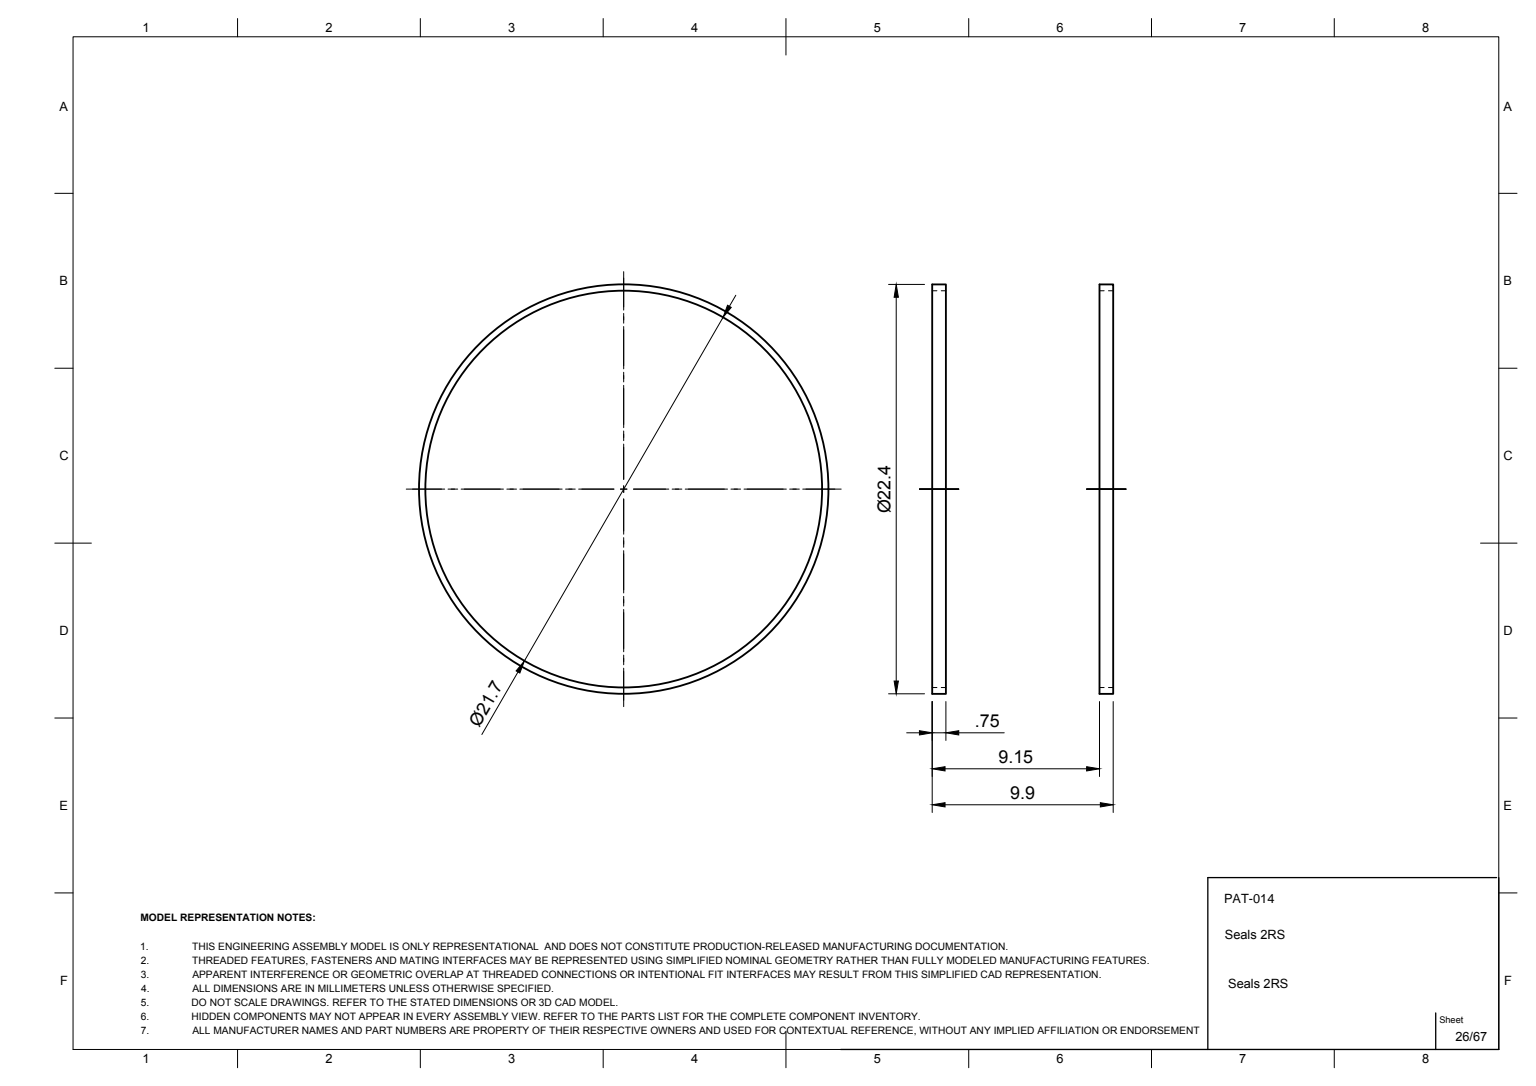
ISO-10303-21;
HEADER;
/* Generated by software containing ST-Developer
 * from STEP Tools, Inc. (www.steptools.com) 
 */

FILE_DESCRIPTION(
/* description */ ('Bin tilter linkage'),
/* implementation_level */ '2;1');

FILE_NAME(
/* name */ 'Seals 2RS.step',
/* time_stamp */ '2026-10-28T03:26:24-07:00',
/* author */ (''),
/* organization */ (''),
/* preprocessor_version */ 'ST-DEVELOPER v20.2',
/* originating_system */ 'Autodesk Translation Framework v15.17.0.0',
/* authorisation */ '');

FILE_SCHEMA (('AUTOMOTIVE_DESIGN { 1 0 10303 214 3 1 1 }'));
ENDSEC;

DATA;
#10=MECHANICAL_DESIGN_GEOMETRIC_PRESENTATION_REPRESENTATION('',(#944,#945),#23728);
#726=SHAPE_REPRESENTATION_RELATIONSHIP('SRR','None',#24193,#832);
#832=ADVANCED_BREP_SHAPE_REPRESENTATION('',(#1057,#1058),#23693);
#944=STYLED_ITEM('',(#24765),#1057);
#945=STYLED_ITEM('',(#24765),#1058);
#1057=MANIFOLD_SOLID_BREP('Body1',#12475);
#1058=MANIFOLD_SOLID_BREP('Body2',#12476);
#1391=FACE_BOUND('',#3517,.T.);
#1392=FACE_BOUND('',#3520,.T.);
#1393=FACE_BOUND('',#3523,.T.);
#1394=FACE_BOUND('',#3526,.T.);
#1749=PLANE('',#14880);
#1750=PLANE('',#14885);
#1751=PLANE('',#14888);
#1752=PLANE('',#14893);
#2435=FACE_OUTER_BOUND('',#3516,.T.);
#2436=FACE_OUTER_BOUND('',#3518,.T.);
#2437=FACE_OUTER_BOUND('',#3519,.T.);
#2438=FACE_OUTER_BOUND('',#3521,.T.);
#2439=FACE_OUTER_BOUND('',#3522,.T.);
#2440=FACE_OUTER_BOUND('',#3524,.T.);
#2441=FACE_OUTER_BOUND('',#3525,.T.);
#2442=FACE_OUTER_BOUND('',#3527,.T.);
#3516=EDGE_LOOP('',(#10387));
#3517=EDGE_LOOP('',(#10388));
#3518=EDGE_LOOP('',(#10389,#10390,#10391,#10392));
#3519=EDGE_LOOP('',(#10393));
#3520=EDGE_LOOP('',(#10394));
#3521=EDGE_LOOP('',(#10395,#10396,#10397,#10398));
#3522=EDGE_LOOP('',(#10399));
#3523=EDGE_LOOP('',(#10400));
#3524=EDGE_LOOP('',(#10401,#10402,#10403,#10404));
#3525=EDGE_LOOP('',(#10405));
#3526=EDGE_LOOP('',(#10406));
#3527=EDGE_LOOP('',(#10407,#10408,#10409,#10410));
#4265=LINE('',#22359,#4940);
#4266=LINE('',#22364,#4941);
#4267=LINE('',#22373,#4942);
#4268=LINE('',#22378,#4943);
#4940=VECTOR('',#18308,1.119765);
#4941=VECTOR('',#18315,1.085235);
#4942=VECTOR('',#18326,1.119765);
#4943=VECTOR('',#18333,1.085235);
#5776=CIRCLE('',#14881,1.119765);
#5777=CIRCLE('',#14882,1.085235);
#5778=CIRCLE('',#14884,1.119765);
#5779=CIRCLE('',#14886,1.085235);
#5780=CIRCLE('',#14889,1.119765);
#5781=CIRCLE('',#14890,1.085235);
#5782=CIRCLE('',#14892,1.119765);
#5783=CIRCLE('',#14894,1.085235);
#6635=VERTEX_POINT('',#22352);
#6636=VERTEX_POINT('',#22354);
#6637=VERTEX_POINT('',#22357);
#6638=VERTEX_POINT('',#22361);
#6639=VERTEX_POINT('',#22366);
#6640=VERTEX_POINT('',#22368);
#6641=VERTEX_POINT('',#22371);
#6642=VERTEX_POINT('',#22375);
#7933=EDGE_CURVE('',#6635,#6635,#5776,.T.);
#7934=EDGE_CURVE('',#6636,#6636,#5777,.T.);
#7935=EDGE_CURVE('',#6637,#6637,#5778,.T.);
#7936=EDGE_CURVE('',#6637,#6635,#4265,.T.);
#7937=EDGE_CURVE('',#6638,#6638,#5779,.T.);
#7938=EDGE_CURVE('',#6638,#6636,#4266,.T.);
#7939=EDGE_CURVE('',#6639,#6639,#5780,.T.);
#7940=EDGE_CURVE('',#6640,#6640,#5781,.T.);
#7941=EDGE_CURVE('',#6641,#6641,#5782,.T.);
#7942=EDGE_CURVE('',#6641,#6639,#4267,.T.);
#7943=EDGE_CURVE('',#6642,#6642,#5783,.T.);
#7944=EDGE_CURVE('',#6642,#6640,#4268,.T.);
#10387=ORIENTED_EDGE('',*,*,#7933,.F.);
#10388=ORIENTED_EDGE('',*,*,#7934,.T.);
#10389=ORIENTED_EDGE('',*,*,#7935,.F.);
#10390=ORIENTED_EDGE('',*,*,#7936,.T.);
#10391=ORIENTED_EDGE('',*,*,#7933,.T.);
#10392=ORIENTED_EDGE('',*,*,#7936,.F.);
#10393=ORIENTED_EDGE('',*,*,#7935,.T.);
#10394=ORIENTED_EDGE('',*,*,#7937,.F.);
#10395=ORIENTED_EDGE('',*,*,#7937,.T.);
#10396=ORIENTED_EDGE('',*,*,#7938,.T.);
#10397=ORIENTED_EDGE('',*,*,#7934,.F.);
#10398=ORIENTED_EDGE('',*,*,#7938,.F.);
#10399=ORIENTED_EDGE('',*,*,#7939,.F.);
#10400=ORIENTED_EDGE('',*,*,#7940,.T.);
#10401=ORIENTED_EDGE('',*,*,#7941,.F.);
#10402=ORIENTED_EDGE('',*,*,#7942,.T.);
#10403=ORIENTED_EDGE('',*,*,#7939,.T.);
#10404=ORIENTED_EDGE('',*,*,#7942,.F.);
#10405=ORIENTED_EDGE('',*,*,#7941,.T.);
#10406=ORIENTED_EDGE('',*,*,#7943,.F.);
#10407=ORIENTED_EDGE('',*,*,#7943,.T.);
#10408=ORIENTED_EDGE('',*,*,#7944,.T.);
#10409=ORIENTED_EDGE('',*,*,#7940,.F.);
#10410=ORIENTED_EDGE('',*,*,#7944,.F.);
#11531=CYLINDRICAL_SURFACE('',#14883,1.119765);
#11532=CYLINDRICAL_SURFACE('',#14887,1.085235);
#11533=CYLINDRICAL_SURFACE('',#14891,1.119765);
#11534=CYLINDRICAL_SURFACE('',#14895,1.085235);
#12160=ADVANCED_FACE('',(#2435,#1391),#1749,.T.);
#12161=ADVANCED_FACE('',(#2436),#11531,.T.);
#12162=ADVANCED_FACE('',(#2437,#1392),#1750,.T.);
#12163=ADVANCED_FACE('',(#2438),#11532,.F.);
#12164=ADVANCED_FACE('',(#2439,#1393),#1751,.T.);
#12165=ADVANCED_FACE('',(#2440),#11533,.T.);
#12166=ADVANCED_FACE('',(#2441,#1394),#1752,.T.);
#12167=ADVANCED_FACE('',(#2442),#11534,.F.);
#12475=CLOSED_SHELL('',(#12160,#12161,#12162,#12163));
#12476=CLOSED_SHELL('',(#12164,#12165,#12166,#12167));
#14879=AXIS2_PLACEMENT_3D('',#22350,#18296,#18297);
#14880=AXIS2_PLACEMENT_3D('',#22351,#18298,#18299);
#14881=AXIS2_PLACEMENT_3D('',#22353,#18300,#18301);
#14882=AXIS2_PLACEMENT_3D('',#22355,#18302,#18303);
#14883=AXIS2_PLACEMENT_3D('',#22356,#18304,#18305);
#14884=AXIS2_PLACEMENT_3D('',#22358,#18306,#18307);
#14885=AXIS2_PLACEMENT_3D('',#22360,#18309,#18310);
#14886=AXIS2_PLACEMENT_3D('',#22362,#18311,#18312);
#14887=AXIS2_PLACEMENT_3D('',#22363,#18313,#18314);
#14888=AXIS2_PLACEMENT_3D('',#22365,#18316,#18317);
#14889=AXIS2_PLACEMENT_3D('',#22367,#18318,#18319);
#14890=AXIS2_PLACEMENT_3D('',#22369,#18320,#18321);
#14891=AXIS2_PLACEMENT_3D('',#22370,#18322,#18323);
#14892=AXIS2_PLACEMENT_3D('',#22372,#18324,#18325);
#14893=AXIS2_PLACEMENT_3D('',#22374,#18327,#18328);
#14894=AXIS2_PLACEMENT_3D('',#22376,#18329,#18330);
#14895=AXIS2_PLACEMENT_3D('',#22377,#18331,#18332);
#18296=DIRECTION('axis',(0.,0.,1.));
#18297=DIRECTION('refdir',(1.,0.,0.));
#18298=DIRECTION('center_axis',(0.,1.,0.));
#18299=DIRECTION('ref_axis',(0.,0.,1.));
#18300=DIRECTION('center_axis',(0.,-1.,0.));
#18301=DIRECTION('ref_axis',(1.,0.,0.));
#18302=DIRECTION('center_axis',(0.,-1.,0.));
#18303=DIRECTION('ref_axis',(1.,0.,0.));
#18304=DIRECTION('center_axis',(0.,-1.,0.));
#18305=DIRECTION('ref_axis',(1.,0.,0.));
#18306=DIRECTION('center_axis',(0.,-1.,0.));
#18307=DIRECTION('ref_axis',(1.,0.,0.));
#18308=DIRECTION('',(0.,1.,0.));
#18309=DIRECTION('center_axis',(0.,-1.,0.));
#18310=DIRECTION('ref_axis',(0.,0.,-1.));
#18311=DIRECTION('center_axis',(0.,-1.,0.));
#18312=DIRECTION('ref_axis',(1.,0.,0.));
#18313=DIRECTION('center_axis',(0.,-1.,0.));
#18314=DIRECTION('ref_axis',(1.,0.,0.));
#18315=DIRECTION('',(0.,1.,0.));
#18316=DIRECTION('center_axis',(0.,1.,0.));
#18317=DIRECTION('ref_axis',(0.,0.,1.));
#18318=DIRECTION('center_axis',(0.,-1.,0.));
#18319=DIRECTION('ref_axis',(1.,0.,0.));
#18320=DIRECTION('center_axis',(0.,-1.,0.));
#18321=DIRECTION('ref_axis',(1.,0.,0.));
#18322=DIRECTION('center_axis',(0.,-1.,0.));
#18323=DIRECTION('ref_axis',(1.,0.,0.));
#18324=DIRECTION('center_axis',(0.,-1.,0.));
#18325=DIRECTION('ref_axis',(1.,0.,0.));
#18326=DIRECTION('',(0.,1.,0.));
#18327=DIRECTION('center_axis',(0.,-1.,0.));
#18328=DIRECTION('ref_axis',(0.,0.,-1.));
#18329=DIRECTION('center_axis',(0.,-1.,0.));
#18330=DIRECTION('ref_axis',(1.,0.,0.));
#18331=DIRECTION('center_axis',(0.,-1.,0.));
#18332=DIRECTION('ref_axis',(1.,0.,0.));
#18333=DIRECTION('',(0.,1.,0.));
#22350=CARTESIAN_POINT('',(0.,0.,0.));
#22351=CARTESIAN_POINT('Origin',(1.119765,0.495,0.));
#22352=CARTESIAN_POINT('',(-1.119765,0.495,-1.37131662304724E-16));
#22353=CARTESIAN_POINT('Origin',(0.,0.495,0.));
#22354=CARTESIAN_POINT('',(-1.085235,0.495,-1.32902956907268E-16));
#22355=CARTESIAN_POINT('Origin',(0.,0.495,0.));
#22356=CARTESIAN_POINT('Origin',(0.,0.4575,0.));
#22357=CARTESIAN_POINT('',(-1.119765,0.42,-1.37131662304724E-16));
#22358=CARTESIAN_POINT('Origin',(0.,0.42,0.));
#22359=CARTESIAN_POINT('',(-1.119765,0.4575,-1.37131662304724E-16));
#22360=CARTESIAN_POINT('Origin',(1.085235,0.42,0.));
#22361=CARTESIAN_POINT('',(-1.085235,0.42,-1.32902956907268E-16));
#22362=CARTESIAN_POINT('Origin',(0.,0.42,0.));
#22363=CARTESIAN_POINT('Origin',(0.,0.4575,0.));
#22364=CARTESIAN_POINT('',(-1.085235,0.4575,-1.32902956907268E-16));
#22365=CARTESIAN_POINT('Origin',(1.119765,-0.42,0.));
#22366=CARTESIAN_POINT('',(-1.119765,-0.42,-1.37131662304724E-16));
#22367=CARTESIAN_POINT('Origin',(0.,-0.42,0.));
#22368=CARTESIAN_POINT('',(-1.085235,-0.42,-1.32902956907268E-16));
#22369=CARTESIAN_POINT('Origin',(0.,-0.42,0.));
#22370=CARTESIAN_POINT('Origin',(0.,-0.4575,0.));
#22371=CARTESIAN_POINT('',(-1.119765,-0.495,-1.37131662304724E-16));
#22372=CARTESIAN_POINT('Origin',(0.,-0.495,0.));
#22373=CARTESIAN_POINT('',(-1.119765,-0.4575,-1.37131662304724E-16));
#22374=CARTESIAN_POINT('Origin',(1.085235,-0.495,0.));
#22375=CARTESIAN_POINT('',(-1.085235,-0.495,-1.32902956907268E-16));
#22376=CARTESIAN_POINT('Origin',(0.,-0.495,0.));
#22377=CARTESIAN_POINT('Origin',(0.,-0.4575,0.));
#22378=CARTESIAN_POINT('',(-1.085235,-0.4575,-1.32902956907268E-16));
#23576=UNCERTAINTY_MEASURE_WITH_UNIT(LENGTH_MEASURE(0.001),#23729,
'DISTANCE_ACCURACY_VALUE',
'Maximum model space distance between geometric entities at asserted c
onnectivities');
#23611=UNCERTAINTY_MEASURE_WITH_UNIT(LENGTH_MEASURE(0.001),#23729,
'DISTANCE_ACCURACY_VALUE',
'Maximum model space distance between geometric entities at asserted c
onnectivities');
#23693=(
GEOMETRIC_REPRESENTATION_CONTEXT(3)
GLOBAL_UNCERTAINTY_ASSIGNED_CONTEXT((#23576))
GLOBAL_UNIT_ASSIGNED_CONTEXT((#23729,#23731,#23732))
REPRESENTATION_CONTEXT('','3D')
);
#23728=(
GEOMETRIC_REPRESENTATION_CONTEXT(3)
GLOBAL_UNCERTAINTY_ASSIGNED_CONTEXT((#23611))
GLOBAL_UNIT_ASSIGNED_CONTEXT((#23729,#23731,#23732))
REPRESENTATION_CONTEXT('','3D')
);
#23729=(
LENGTH_UNIT()
NAMED_UNIT(*)
SI_UNIT(.CENTI.,.METRE.)
);
#23731=(
NAMED_UNIT(*)
PLANE_ANGLE_UNIT()
SI_UNIT($,.RADIAN.)
);
#23732=(
NAMED_UNIT(*)
SI_UNIT($,.STERADIAN.)
SOLID_ANGLE_UNIT()
);
#23814=SHAPE_DEFINITION_REPRESENTATION(#23930,#24193);
#23930=PRODUCT_DEFINITION_SHAPE('',$,#24310);
#24193=SHAPE_REPRESENTATION('',(#14879),#23693);
#24228=PRODUCT_DEFINITION_CONTEXT('part definition',#24578,'design');
#24310=PRODUCT_DEFINITION('Seals 2RS','Seals 2RS',#24426,#24228);
#24426=PRODUCT_DEFINITION_FORMATION('',$,#24661);
#24578=APPLICATION_CONTEXT(
'Core Data for Automotive Mechanical Design Process');
#24579=PRODUCT_CONTEXT('part definition',#24578,'mechanical');
#24661=PRODUCT('Seals 2RS','Seals 2RS','Seals 2RS',(#24579));
#24759=COLOUR_RGB('Grey',0.48,0.52,0.57);
#24760=FILL_AREA_STYLE_COLOUR('',#24759);
#24761=FILL_AREA_STYLE('',(#24760));
#24762=SURFACE_STYLE_FILL_AREA(#24761);
#24763=SURFACE_SIDE_STYLE('',(#24762));
#24764=SURFACE_STYLE_USAGE(.BOTH.,#24763);
#24765=PRESENTATION_STYLE_ASSIGNMENT((#24764));
ENDSEC;
END-ISO-10303-21;
